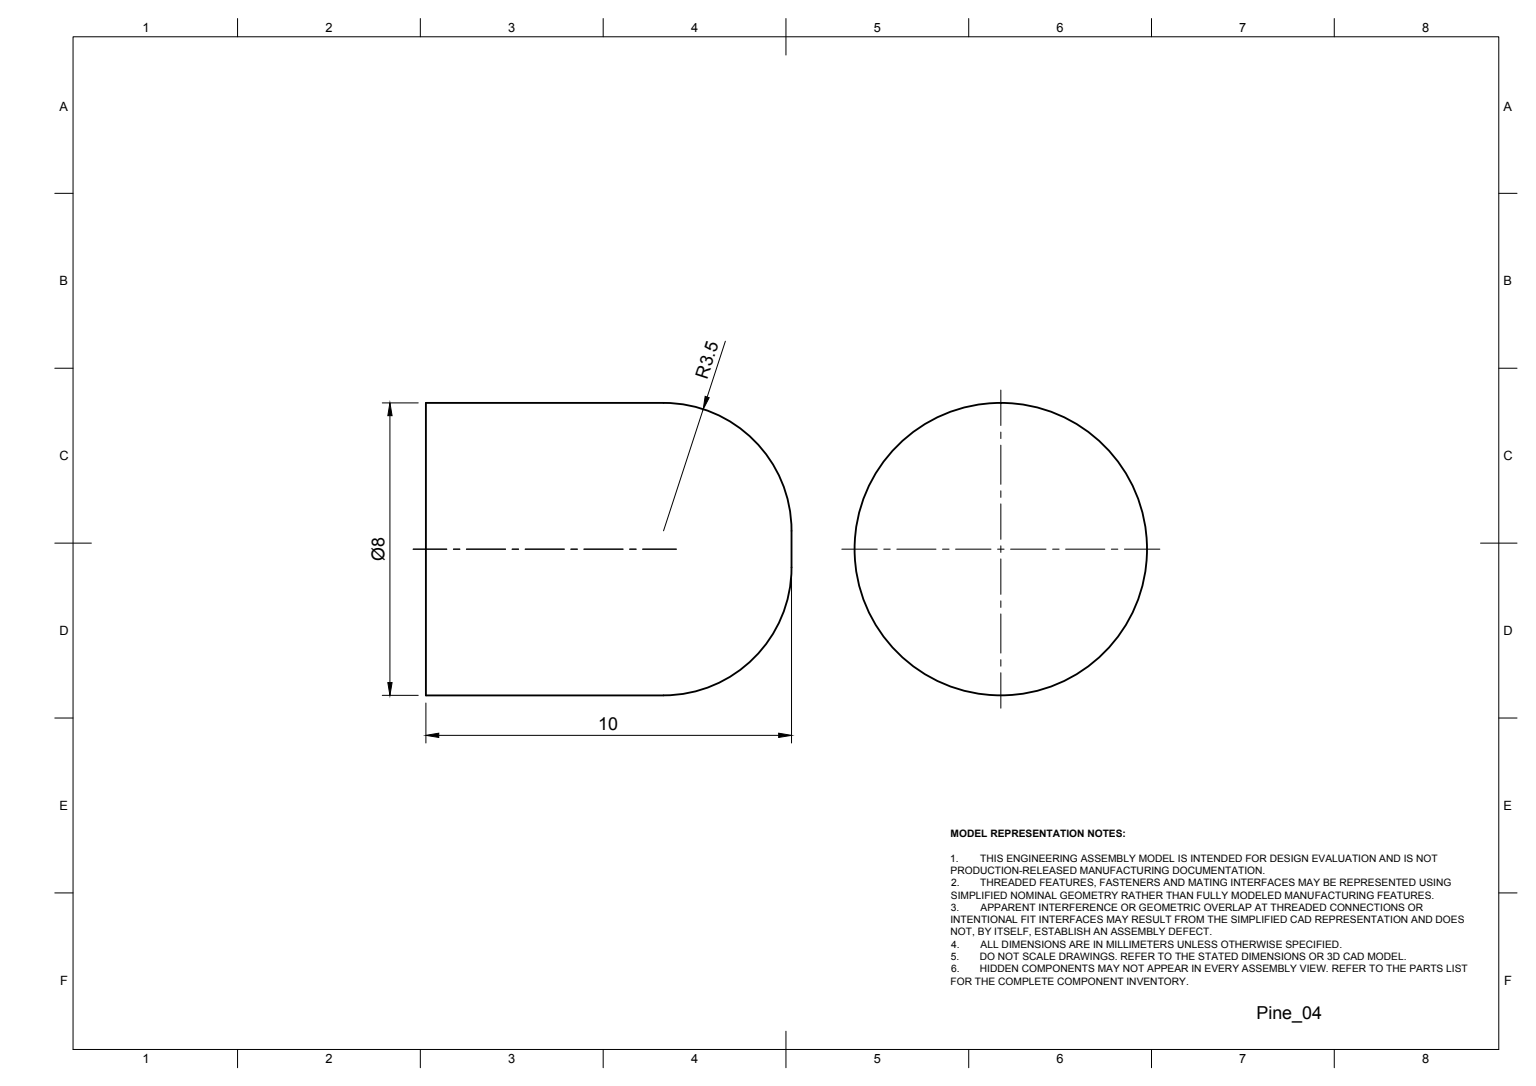
ISO-10303-21;
HEADER;
/* Generated by software containing ST-Developer
 * from STEP Tools, Inc. (www.steptools.com) 
 */

FILE_DESCRIPTION(
/* description */ (''),
/* implementation_level */ '2;1');

FILE_NAME(
/* name */ 'Pine_04.step',
/* time_stamp */ '2026-10-06T13:31:15-07:00',
/* author */ (''),
/* organization */ (''),
/* preprocessor_version */ 'ST-DEVELOPER v20.2',
/* originating_system */ 'Autodesk Translation Framework v15.15.0.0',
/* authorisation */ '');

FILE_SCHEMA (('AUTOMOTIVE_DESIGN { 1 0 10303 214 3 1 1 }'));
ENDSEC;

DATA;
#10=MECHANICAL_DESIGN_GEOMETRIC_PRESENTATION_REPRESENTATION('',(#82),#3154);
#47=(
BOUNDED_SURFACE()
B_SPLINE_SURFACE(2,2,((#2142,#2143,#2144,#2145,#2146,#2147,#2148,#2149,
#2150),(#2151,#2152,#2153,#2154,#2155,#2156,#2157,#2158,#2159),(#2160,#2161,
#2162,#2163,#2164,#2165,#2166,#2167,#2168)),.UNSPECIFIED.,.F.,.T.,.F.)
B_SPLINE_SURFACE_WITH_KNOTS((3,3),(3,2,2,2,3),(-1.57079632679497,6.11109985317371E-14),
(-3.14159265358979,-1.5707963267949,0.,1.5707963267949,3.14159265358979),
 .UNSPECIFIED.)
GEOMETRIC_REPRESENTATION_ITEM()
RATIONAL_B_SPLINE_SURFACE(((1.,0.707106781186548,1.,0.707106781186548,1.,
0.707106781186548,1.,0.707106781186548,1.),(0.707106781186505,0.49999999999997,
0.707106781186505,0.49999999999997,0.707106781186505,0.49999999999997,0.707106781186505,
0.49999999999997,0.707106781186505),(1.,0.707106781186548,1.,0.707106781186548,
1.,0.707106781186548,1.,0.707106781186548,1.)))
REPRESENTATION_ITEM('')
SURFACE()
);
#64=SHAPE_REPRESENTATION_RELATIONSHIP('SRR','None',#3192,#73);
#73=ADVANCED_BREP_SHAPE_REPRESENTATION('',(#91),#3148);
#82=STYLED_ITEM('',(#3243),#91);
#91=MANIFOLD_SOLID_BREP('Body1',#1084);
#110=PLANE('',#1228);
#111=PLANE('',#1229);
#147=CIRCLE('',#1222,3.99999999999999);
#148=CIRCLE('',#1223,3.99999999999999);
#149=CIRCLE('',#1224,3.49999999999999);
#150=CIRCLE('',#1225,0.49999999999999);
#151=CIRCLE('',#1227,3.99999999999999);
#194=FACE_OUTER_BOUND('',#258,.T.);
#195=FACE_OUTER_BOUND('',#259,.T.);
#196=FACE_OUTER_BOUND('',#260,.T.);
#197=FACE_OUTER_BOUND('',#261,.T.);
#258=EDGE_LOOP('',(#832,#833,#834,#835,#836));
#259=EDGE_LOOP('',(#837,#838,#839,#840,#841));
#260=EDGE_LOOP('',(#842));
#261=EDGE_LOOP('',(#843));
#330=LINE('',#2179,#396);
#396=VECTOR('',#1392,3.99999999999999);
#516=VERTEX_POINT('',#2169);
#517=VERTEX_POINT('',#2170);
#518=VERTEX_POINT('',#2173);
#519=VERTEX_POINT('',#2177);
#632=EDGE_CURVE('',#516,#517,#147,.T.);
#633=EDGE_CURVE('',#517,#516,#148,.T.);
#634=EDGE_CURVE('',#517,#518,#149,.T.);
#635=EDGE_CURVE('',#518,#518,#150,.T.);
#636=EDGE_CURVE('',#519,#519,#151,.T.);
#637=EDGE_CURVE('',#519,#516,#330,.T.);
#832=ORIENTED_EDGE('',*,*,#632,.F.);
#833=ORIENTED_EDGE('',*,*,#633,.F.);
#834=ORIENTED_EDGE('',*,*,#634,.T.);
#835=ORIENTED_EDGE('',*,*,#635,.F.);
#836=ORIENTED_EDGE('',*,*,#634,.F.);
#837=ORIENTED_EDGE('',*,*,#636,.F.);
#838=ORIENTED_EDGE('',*,*,#637,.T.);
#839=ORIENTED_EDGE('',*,*,#632,.T.);
#840=ORIENTED_EDGE('',*,*,#633,.T.);
#841=ORIENTED_EDGE('',*,*,#637,.F.);
#842=ORIENTED_EDGE('',*,*,#635,.T.);
#843=ORIENTED_EDGE('',*,*,#636,.T.);
#1014=CYLINDRICAL_SURFACE('',#1226,3.99999999999999);
#1045=ADVANCED_FACE('',(#194),#47,.F.);
#1046=ADVANCED_FACE('',(#195),#1014,.T.);
#1047=ADVANCED_FACE('',(#196),#110,.F.);
#1048=ADVANCED_FACE('',(#197),#111,.T.);
#1084=CLOSED_SHELL('',(#1045,#1046,#1047,#1048));
#1221=AXIS2_PLACEMENT_3D('',#2141,#1378,#1379);
#1222=AXIS2_PLACEMENT_3D('',#2171,#1380,#1381);
#1223=AXIS2_PLACEMENT_3D('',#2172,#1382,#1383);
#1224=AXIS2_PLACEMENT_3D('',#2174,#1384,#1385);
#1225=AXIS2_PLACEMENT_3D('',#2175,#1386,#1387);
#1226=AXIS2_PLACEMENT_3D('',#2176,#1388,#1389);
#1227=AXIS2_PLACEMENT_3D('',#2178,#1390,#1391);
#1228=AXIS2_PLACEMENT_3D('',#2180,#1393,#1394);
#1229=AXIS2_PLACEMENT_3D('',#2181,#1395,#1396);
#1378=DIRECTION('axis',(0.,0.,1.));
#1379=DIRECTION('refdir',(1.,0.,0.));
#1380=DIRECTION('center_axis',(1.,0.,0.));
#1381=DIRECTION('ref_axis',(0.,1.,0.));
#1382=DIRECTION('center_axis',(1.,0.,0.));
#1383=DIRECTION('ref_axis',(0.,1.,0.));
#1384=DIRECTION('center_axis',(-5.11592739497909E-14,-1.,-1.22464679913998E-16));
#1385=DIRECTION('ref_axis',(1.44328993201271E-14,-1.22464679914736E-16,
1.));
#1386=DIRECTION('center_axis',(-1.,0.,0.));
#1387=DIRECTION('ref_axis',(0.,1.,0.));
#1388=DIRECTION('center_axis',(1.,0.,0.));
#1389=DIRECTION('ref_axis',(0.,1.,0.));
#1390=DIRECTION('center_axis',(1.,0.,0.));
#1391=DIRECTION('ref_axis',(0.,1.,0.));
#1392=DIRECTION('',(-1.,0.,0.));
#1393=DIRECTION('center_axis',(1.,0.,0.));
#1394=DIRECTION('ref_axis',(0.,1.,0.));
#1395=DIRECTION('center_axis',(1.,0.,0.));
#1396=DIRECTION('ref_axis',(0.,1.,0.));
#2141=CARTESIAN_POINT('',(0.,0.,0.));
#2142=CARTESIAN_POINT('Ctrl Pts',(-27.,1.99568395523348E-13,320.5));
#2143=CARTESIAN_POINT('Ctrl Pts',(-27.,-0.499999999999559,320.5));
#2144=CARTESIAN_POINT('Ctrl Pts',(-27.,-0.499999999999559,320.));
#2145=CARTESIAN_POINT('Ctrl Pts',(-27.,-0.499999999999559,319.5));
#2146=CARTESIAN_POINT('Ctrl Pts',(-27.,1.99568395523348E-13,319.5));
#2147=CARTESIAN_POINT('Ctrl Pts',(-27.,0.499999999999958,319.5));
#2148=CARTESIAN_POINT('Ctrl Pts',(-27.,0.499999999999958,320.));
#2149=CARTESIAN_POINT('Ctrl Pts',(-26.9999999999999,0.499999999999958,320.5));
#2150=CARTESIAN_POINT('Ctrl Pts',(-27.,1.99568395523348E-13,320.5));
#2151=CARTESIAN_POINT('Ctrl Pts',(-27.0000000000002,1.99568395523362E-13,
324.));
#2152=CARTESIAN_POINT('Ctrl Pts',(-27.0000000000004,-4.00000000000003,324.));
#2153=CARTESIAN_POINT('Ctrl Pts',(-27.0000000000004,-4.00000000000003,320.));
#2154=CARTESIAN_POINT('Ctrl Pts',(-27.0000000000005,-4.00000000000003,316.));
#2155=CARTESIAN_POINT('Ctrl Pts',(-27.0000000000003,1.99568395523362E-13,
316.));
#2156=CARTESIAN_POINT('Ctrl Pts',(-27.0000000000001,4.00000000000043,316.));
#2157=CARTESIAN_POINT('Ctrl Pts',(-27.,4.00000000000043,320.));
#2158=CARTESIAN_POINT('Ctrl Pts',(-27.,4.00000000000043,324.));
#2159=CARTESIAN_POINT('Ctrl Pts',(-27.0000000000002,1.99568395523362E-13,
324.));
#2160=CARTESIAN_POINT('Ctrl Pts',(-23.4999999999997,2.05109366990699E-14,
324.));
#2161=CARTESIAN_POINT('Ctrl Pts',(-23.4999999999999,-3.99999999999996,324.));
#2162=CARTESIAN_POINT('Ctrl Pts',(-23.5,-3.99999999999997,320.));
#2163=CARTESIAN_POINT('Ctrl Pts',(-23.5,-3.99999999999996,316.));
#2164=CARTESIAN_POINT('Ctrl Pts',(-23.4999999999998,2.05109366990698E-14,
316.));
#2165=CARTESIAN_POINT('Ctrl Pts',(-23.4999999999996,4.00000000000001,316.));
#2166=CARTESIAN_POINT('Ctrl Pts',(-23.4999999999996,4.00000000000001,320.));
#2167=CARTESIAN_POINT('Ctrl Pts',(-23.4999999999995,4.00000000000001,324.));
#2168=CARTESIAN_POINT('Ctrl Pts',(-23.4999999999997,2.05109366990699E-14,
324.));
#2169=CARTESIAN_POINT('',(-23.5,-3.99999999999999,320.));
#2170=CARTESIAN_POINT('',(-23.5,2.00210779794253E-14,324.));
#2171=CARTESIAN_POINT('Origin',(-23.5,0.,320.));
#2172=CARTESIAN_POINT('Origin',(-23.5,0.,320.));
#2173=CARTESIAN_POINT('',(-27.,-6.12323399573687E-17,320.5));
#2174=CARTESIAN_POINT('Origin',(-23.5,2.04497043591234E-14,320.5));
#2175=CARTESIAN_POINT('Origin',(-27.,0.,320.));
#2176=CARTESIAN_POINT('Origin',(-2.,0.,320.));
#2177=CARTESIAN_POINT('',(-17.,-3.99999999999999,320.));
#2178=CARTESIAN_POINT('Origin',(-17.,0.,320.));
#2179=CARTESIAN_POINT('',(-2.,-3.99999999999999,320.));
#2180=CARTESIAN_POINT('Origin',(-27.,0.,320.));
#2181=CARTESIAN_POINT('Origin',(-17.,0.,320.));
#3137=UNCERTAINTY_MEASURE_WITH_UNIT(LENGTH_MEASURE(0.01),#3155,
'DISTANCE_ACCURACY_VALUE',
'Maximum model space distance between geometric entities at asserted c
onnectivities');
#3143=UNCERTAINTY_MEASURE_WITH_UNIT(LENGTH_MEASURE(0.01),#3155,
'DISTANCE_ACCURACY_VALUE',
'Maximum model space distance between geometric entities at asserted c
onnectivities');
#3148=(
GEOMETRIC_REPRESENTATION_CONTEXT(3)
GLOBAL_UNCERTAINTY_ASSIGNED_CONTEXT((#3137))
GLOBAL_UNIT_ASSIGNED_CONTEXT((#3155,#3157,#3158))
REPRESENTATION_CONTEXT('','3D')
);
#3154=(
GEOMETRIC_REPRESENTATION_CONTEXT(3)
GLOBAL_UNCERTAINTY_ASSIGNED_CONTEXT((#3143))
GLOBAL_UNIT_ASSIGNED_CONTEXT((#3155,#3157,#3158))
REPRESENTATION_CONTEXT('','3D')
);
#3155=(
LENGTH_UNIT()
NAMED_UNIT(*)
SI_UNIT(.MILLI.,.METRE.)
);
#3157=(
NAMED_UNIT(*)
PLANE_ANGLE_UNIT()
SI_UNIT($,.RADIAN.)
);
#3158=(
NAMED_UNIT(*)
SI_UNIT($,.STERADIAN.)
SOLID_ANGLE_UNIT()
);
#3163=SHAPE_DEFINITION_REPRESENTATION(#3173,#3192);
#3173=PRODUCT_DEFINITION_SHAPE('',$,#3203);
#3192=SHAPE_REPRESENTATION('',(#1221),#3148);
#3198=PRODUCT_DEFINITION_CONTEXT('part definition',#3230,'design');
#3203=PRODUCT_DEFINITION('Pine_04','Pine_04',#3213,#3198);
#3213=PRODUCT_DEFINITION_FORMATION('',$,#3236);
#3230=APPLICATION_CONTEXT(
'Core Data for Automotive Mechanical Design Process');
#3231=PRODUCT_CONTEXT('part definition',#3230,'mechanical');
#3236=PRODUCT('Pine_04','Pine_04',$,(#3231));
#3243=PRESENTATION_STYLE_ASSIGNMENT((#3245));
#3245=SURFACE_STYLE_USAGE(.BOTH.,#3247);
#3247=SURFACE_SIDE_STYLE('',(#3249));
#3249=SURFACE_STYLE_FILL_AREA(#3251);
#3251=FILL_AREA_STYLE('Opaque(160,160,160)',(#3253));
#3253=FILL_AREA_STYLE_COLOUR('Opaque(160,160,160)',#3255);
#3255=COLOUR_RGB('Opaque(160,160,160)', 0.09019608, 0.27058824, 0.51372549);
ENDSEC;
END-ISO-10303-21;
